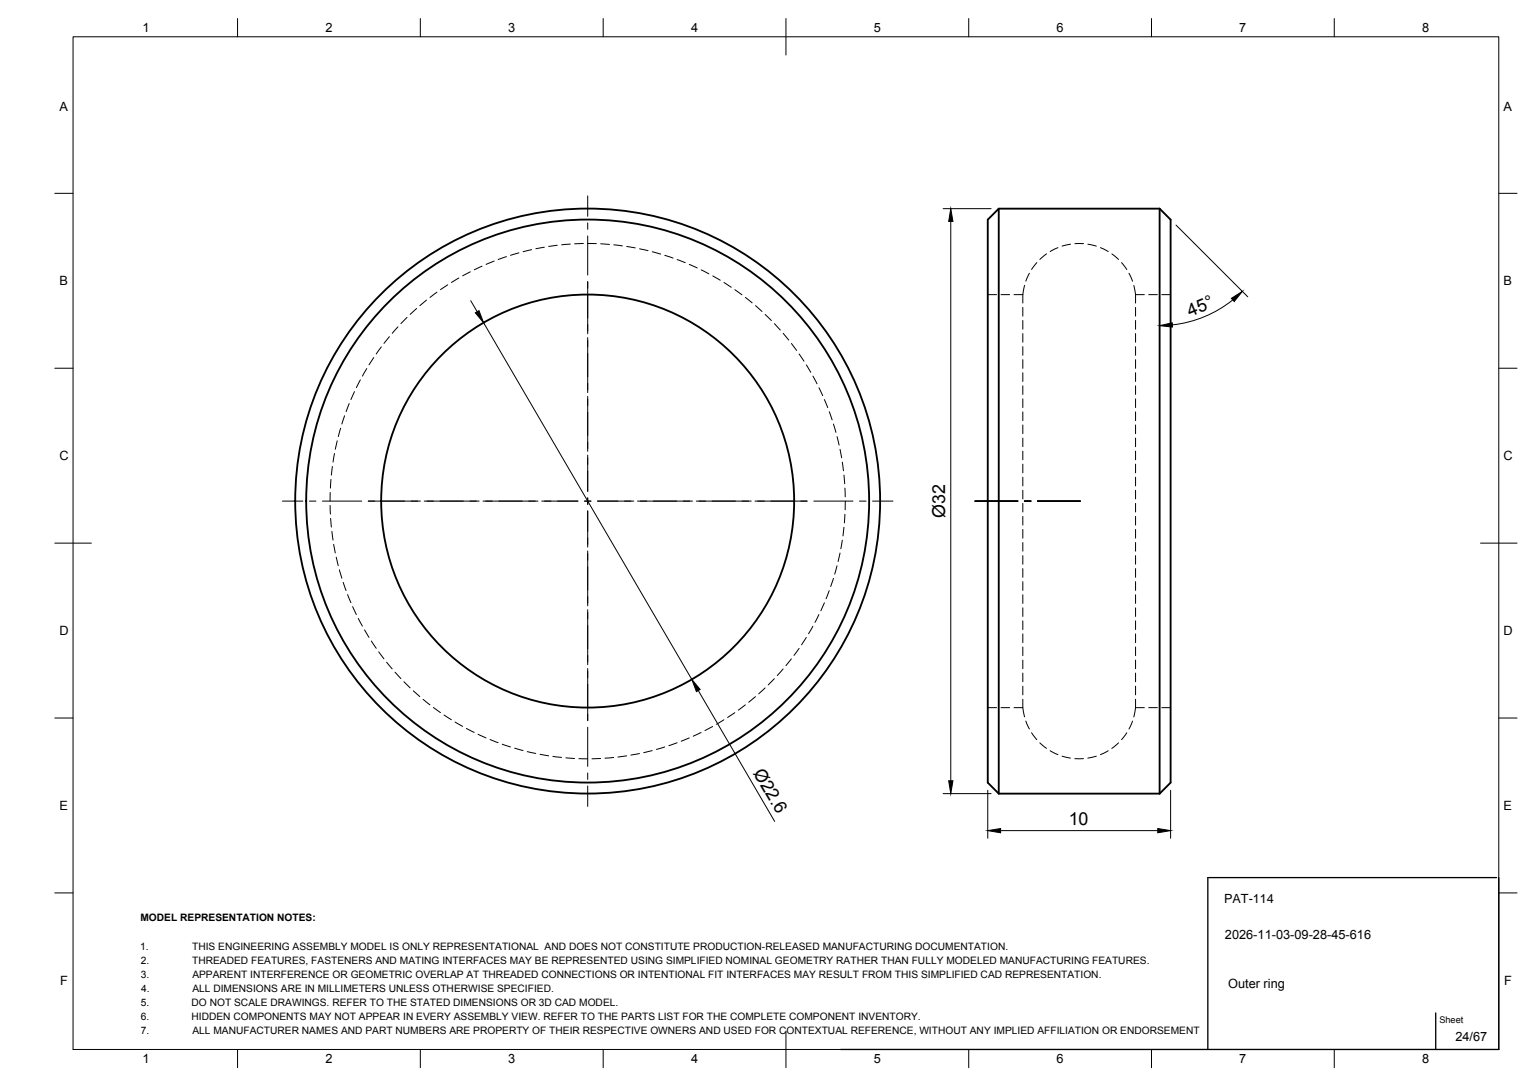
ISO-10303-21;
HEADER;
/* Generated by software containing ST-Developer
 * from STEP Tools, Inc. (www.steptools.com) 
 */

FILE_DESCRIPTION(
/* description */ ('Two-stage gear reducer in split housing'),
/* implementation_level */ '2;1');

FILE_NAME(
/* name */ 'Outer ring.step',
/* time_stamp */ '2026-10-28T03:22:31-07:00',
/* author */ (''),
/* organization */ (''),
/* preprocessor_version */ 'ST-DEVELOPER v20.2',
/* originating_system */ 'Autodesk Translation Framework v15.17.0.0',
/* authorisation */ '');

FILE_SCHEMA (('AUTOMOTIVE_DESIGN { 1 0 10303 214 3 1 1 }'));
ENDSEC;

DATA;
#10=MECHANICAL_DESIGN_GEOMETRIC_PRESENTATION_REPRESENTATION('',(#1252),#73366);
#1098=TOROIDAL_SURFACE('',#17438,1.1,0.309556);
#1106=CONICAL_SURFACE('',#17449,1.57,0.785398163397449);
#1107=CONICAL_SURFACE('',#17453,1.57,0.785398163397449);
#1140=SHAPE_REPRESENTATION_RELATIONSHIP('SRR','None',#73628,#1196);
#1196=ADVANCED_BREP_SHAPE_REPRESENTATION('',(#1322),#73324);
#1252=STYLED_ITEM('',(#73988),#1322);
#1322=MANIFOLD_SOLID_BREP('Body1',#16141);
#1521=FACE_BOUND('',#3371,.T.);
#1522=FACE_BOUND('',#3376,.T.);
#1757=PLANE('',#17446);
#1758=PLANE('',#17455);
#2308=FACE_OUTER_BOUND('',#3368,.T.);
#2309=FACE_OUTER_BOUND('',#3369,.T.);
#2310=FACE_OUTER_BOUND('',#3370,.T.);
#2311=FACE_OUTER_BOUND('',#3372,.T.);
#2312=FACE_OUTER_BOUND('',#3373,.T.);
#2313=FACE_OUTER_BOUND('',#3374,.T.);
#2314=FACE_OUTER_BOUND('',#3375,.T.);
#2315=FACE_OUTER_BOUND('',#3377,.T.);
#3368=EDGE_LOOP('',(#11847,#11848,#11849,#11850,#11851,#11852));
#3369=EDGE_LOOP('',(#11853,#11854,#11855,#11856,#11857));
#3370=EDGE_LOOP('',(#11858));
#3371=EDGE_LOOP('',(#11859));
#3372=EDGE_LOOP('',(#11860,#11861,#11862,#11863));
#3373=EDGE_LOOP('',(#11864,#11865,#11866,#11867));
#3374=EDGE_LOOP('',(#11868,#11869,#11870,#11871));
#3375=EDGE_LOOP('',(#11872));
#3376=EDGE_LOOP('',(#11873));
#3377=EDGE_LOOP('',(#11874,#11875,#11876,#11877,#11878));
#4428=LINE('',#24230,#5452);
#4429=LINE('',#24239,#5453);
#4430=LINE('',#24243,#5454);
#4431=LINE('',#24247,#5455);
#4432=LINE('',#24250,#5456);
#5452=VECTOR('',#20098,1.129765);
#5453=VECTOR('',#20109,1.57);
#5454=VECTOR('',#20114,1.6);
#5455=VECTOR('',#20119,1.57);
#5456=VECTOR('',#20124,1.129765);
#6402=CIRCLE('',#17439,1.129765);
#6403=CIRCLE('',#17440,1.129765);
#6404=CIRCLE('',#17441,0.309556);
#6405=CIRCLE('',#17442,1.129765);
#6406=CIRCLE('',#17443,1.129765);
#6407=CIRCLE('',#17445,1.129765);
#6408=CIRCLE('',#17447,1.54);
#6409=CIRCLE('',#17448,1.129765);
#6410=CIRCLE('',#17450,1.6);
#6411=CIRCLE('',#17452,1.6);
#6412=CIRCLE('',#17454,1.54);
#7269=VERTEX_POINT('',#24218);
#7270=VERTEX_POINT('',#24219);
#7271=VERTEX_POINT('',#24222);
#7272=VERTEX_POINT('',#24224);
#7273=VERTEX_POINT('',#24228);
#7274=VERTEX_POINT('',#24232);
#7275=VERTEX_POINT('',#24234);
#7276=VERTEX_POINT('',#24237);
#7277=VERTEX_POINT('',#24241);
#7278=VERTEX_POINT('',#24245);
#8977=EDGE_CURVE('',#7269,#7270,#6402,.T.);
#8978=EDGE_CURVE('',#7270,#7269,#6403,.T.);
#8979=EDGE_CURVE('',#7270,#7271,#6404,.T.);
#8980=EDGE_CURVE('',#7272,#7271,#6405,.T.);
#8981=EDGE_CURVE('',#7271,#7272,#6406,.T.);
#8982=EDGE_CURVE('',#7273,#7273,#6407,.T.);
#8983=EDGE_CURVE('',#7273,#7272,#4428,.T.);
#8984=EDGE_CURVE('',#7274,#7274,#6408,.T.);
#8985=EDGE_CURVE('',#7275,#7275,#6409,.T.);
#8986=EDGE_CURVE('',#7276,#7276,#6410,.T.);
#8987=EDGE_CURVE('',#7276,#7274,#4429,.T.);
#8988=EDGE_CURVE('',#7277,#7277,#6411,.T.);
#8989=EDGE_CURVE('',#7277,#7276,#4430,.T.);
#8990=EDGE_CURVE('',#7278,#7278,#6412,.T.);
#8991=EDGE_CURVE('',#7278,#7277,#4431,.T.);
#8992=EDGE_CURVE('',#7269,#7275,#4432,.T.);
#11847=ORIENTED_EDGE('',*,*,#8977,.F.);
#11848=ORIENTED_EDGE('',*,*,#8978,.F.);
#11849=ORIENTED_EDGE('',*,*,#8979,.T.);
#11850=ORIENTED_EDGE('',*,*,#8980,.F.);
#11851=ORIENTED_EDGE('',*,*,#8981,.F.);
#11852=ORIENTED_EDGE('',*,*,#8979,.F.);
#11853=ORIENTED_EDGE('',*,*,#8982,.T.);
#11854=ORIENTED_EDGE('',*,*,#8983,.T.);
#11855=ORIENTED_EDGE('',*,*,#8980,.T.);
#11856=ORIENTED_EDGE('',*,*,#8981,.T.);
#11857=ORIENTED_EDGE('',*,*,#8983,.F.);
#11858=ORIENTED_EDGE('',*,*,#8984,.F.);
#11859=ORIENTED_EDGE('',*,*,#8985,.T.);
#11860=ORIENTED_EDGE('',*,*,#8986,.F.);
#11861=ORIENTED_EDGE('',*,*,#8987,.T.);
#11862=ORIENTED_EDGE('',*,*,#8984,.T.);
#11863=ORIENTED_EDGE('',*,*,#8987,.F.);
#11864=ORIENTED_EDGE('',*,*,#8988,.F.);
#11865=ORIENTED_EDGE('',*,*,#8989,.T.);
#11866=ORIENTED_EDGE('',*,*,#8986,.T.);
#11867=ORIENTED_EDGE('',*,*,#8989,.F.);
#11868=ORIENTED_EDGE('',*,*,#8990,.F.);
#11869=ORIENTED_EDGE('',*,*,#8991,.T.);
#11870=ORIENTED_EDGE('',*,*,#8988,.T.);
#11871=ORIENTED_EDGE('',*,*,#8991,.F.);
#11872=ORIENTED_EDGE('',*,*,#8990,.T.);
#11873=ORIENTED_EDGE('',*,*,#8982,.F.);
#11874=ORIENTED_EDGE('',*,*,#8977,.T.);
#11875=ORIENTED_EDGE('',*,*,#8978,.T.);
#11876=ORIENTED_EDGE('',*,*,#8992,.T.);
#11877=ORIENTED_EDGE('',*,*,#8985,.F.);
#11878=ORIENTED_EDGE('',*,*,#8992,.F.);
#15052=CYLINDRICAL_SURFACE('',#17444,1.129765);
#15053=CYLINDRICAL_SURFACE('',#17451,1.6);
#15054=CYLINDRICAL_SURFACE('',#17456,1.129765);
#15515=ADVANCED_FACE('',(#2308),#1098,.F.);
#15516=ADVANCED_FACE('',(#2309),#15052,.F.);
#15517=ADVANCED_FACE('',(#2310,#1521),#1757,.T.);
#15518=ADVANCED_FACE('',(#2311),#1106,.T.);
#15519=ADVANCED_FACE('',(#2312),#15053,.T.);
#15520=ADVANCED_FACE('',(#2313),#1107,.T.);
#15521=ADVANCED_FACE('',(#2314,#1522),#1758,.T.);
#15522=ADVANCED_FACE('',(#2315),#15054,.F.);
#16141=CLOSED_SHELL('',(#15515,#15516,#15517,#15518,#15519,#15520,#15521,
#15522));
#17437=AXIS2_PLACEMENT_3D('',#24216,#20080,#20081);
#17438=AXIS2_PLACEMENT_3D('',#24217,#20082,#20083);
#17439=AXIS2_PLACEMENT_3D('',#24220,#20084,#20085);
#17440=AXIS2_PLACEMENT_3D('',#24221,#20086,#20087);
#17441=AXIS2_PLACEMENT_3D('',#24223,#20088,#20089);
#17442=AXIS2_PLACEMENT_3D('',#24225,#20090,#20091);
#17443=AXIS2_PLACEMENT_3D('',#24226,#20092,#20093);
#17444=AXIS2_PLACEMENT_3D('',#24227,#20094,#20095);
#17445=AXIS2_PLACEMENT_3D('',#24229,#20096,#20097);
#17446=AXIS2_PLACEMENT_3D('',#24231,#20099,#20100);
#17447=AXIS2_PLACEMENT_3D('',#24233,#20101,#20102);
#17448=AXIS2_PLACEMENT_3D('',#24235,#20103,#20104);
#17449=AXIS2_PLACEMENT_3D('',#24236,#20105,#20106);
#17450=AXIS2_PLACEMENT_3D('',#24238,#20107,#20108);
#17451=AXIS2_PLACEMENT_3D('',#24240,#20110,#20111);
#17452=AXIS2_PLACEMENT_3D('',#24242,#20112,#20113);
#17453=AXIS2_PLACEMENT_3D('',#24244,#20115,#20116);
#17454=AXIS2_PLACEMENT_3D('',#24246,#20117,#20118);
#17455=AXIS2_PLACEMENT_3D('',#24248,#20120,#20121);
#17456=AXIS2_PLACEMENT_3D('',#24249,#20122,#20123);
#20080=DIRECTION('axis',(0.,0.,1.));
#20081=DIRECTION('refdir',(1.,0.,0.));
#20082=DIRECTION('center_axis',(0.,-1.,0.));
#20083=DIRECTION('ref_axis',(0.,0.,-1.));
#20084=DIRECTION('center_axis',(0.,-1.,0.));
#20085=DIRECTION('ref_axis',(1.,0.,0.));
#20086=DIRECTION('center_axis',(0.,-1.,0.));
#20087=DIRECTION('ref_axis',(1.,0.,0.));
#20088=DIRECTION('center_axis',(1.,0.,1.22464679914735E-16));
#20089=DIRECTION('ref_axis',(-1.22464679914735E-16,0.,1.));
#20090=DIRECTION('center_axis',(0.,1.,0.));
#20091=DIRECTION('ref_axis',(1.,0.,0.));
#20092=DIRECTION('center_axis',(0.,1.,0.));
#20093=DIRECTION('ref_axis',(1.,0.,0.));
#20094=DIRECTION('center_axis',(0.,-1.,0.));
#20095=DIRECTION('ref_axis',(1.,0.,0.));
#20096=DIRECTION('center_axis',(0.,-1.,0.));
#20097=DIRECTION('ref_axis',(1.,0.,0.));
#20098=DIRECTION('',(0.,1.,0.));
#20099=DIRECTION('center_axis',(0.,1.,0.));
#20100=DIRECTION('ref_axis',(0.,0.,1.));
#20101=DIRECTION('center_axis',(0.,-1.,0.));
#20102=DIRECTION('ref_axis',(1.,0.,0.));
#20103=DIRECTION('center_axis',(0.,-1.,0.));
#20104=DIRECTION('ref_axis',(1.,0.,0.));
#20105=DIRECTION('center_axis',(0.,-1.,0.));
#20106=DIRECTION('ref_axis',(1.,0.,0.));
#20107=DIRECTION('center_axis',(0.,-1.,0.));
#20108=DIRECTION('ref_axis',(1.,0.,0.));
#20109=DIRECTION('',(0.707106781186548,0.707106781186547,8.65956056235494E-17));
#20110=DIRECTION('center_axis',(0.,-1.,0.));
#20111=DIRECTION('ref_axis',(1.,0.,0.));
#20112=DIRECTION('center_axis',(0.,-1.,0.));
#20113=DIRECTION('ref_axis',(1.,0.,0.));
#20114=DIRECTION('',(0.,1.,0.));
#20115=DIRECTION('center_axis',(0.,1.,0.));
#20116=DIRECTION('ref_axis',(1.,0.,0.));
#20117=DIRECTION('center_axis',(0.,-1.,0.));
#20118=DIRECTION('ref_axis',(1.,0.,0.));
#20119=DIRECTION('',(-0.707106781186548,0.707106781186547,-8.65956056235494E-17));
#20120=DIRECTION('center_axis',(0.,-1.,0.));
#20121=DIRECTION('ref_axis',(0.,0.,-1.));
#20122=DIRECTION('center_axis',(0.,-1.,0.));
#20123=DIRECTION('ref_axis',(1.,0.,0.));
#20124=DIRECTION('',(0.,1.,0.));
#24216=CARTESIAN_POINT('',(0.,0.,0.));
#24217=CARTESIAN_POINT('Origin',(0.,0.,0.));
#24218=CARTESIAN_POINT('',(-1.129765,0.308121667383195,-1.38356309103871E-16));
#24219=CARTESIAN_POINT('',(-1.38356309103871E-16,0.308121667383195,1.129765));
#24220=CARTESIAN_POINT('Origin',(0.,0.308121667383195,0.));
#24221=CARTESIAN_POINT('Origin',(0.,0.308121667383195,0.));
#24222=CARTESIAN_POINT('',(-1.38356309103871E-16,-0.308121667383195,1.129765));
#24223=CARTESIAN_POINT('Origin',(-1.34711147906209E-16,0.,1.1));
#24224=CARTESIAN_POINT('',(-1.129765,-0.308121667383195,1.38356309103871E-16));
#24225=CARTESIAN_POINT('Origin',(0.,-0.308121667383195,0.));
#24226=CARTESIAN_POINT('Origin',(0.,-0.308121667383195,0.));
#24227=CARTESIAN_POINT('Origin',(0.,0.,0.));
#24228=CARTESIAN_POINT('',(-1.129765,-0.5,-1.38356309103871E-16));
#24229=CARTESIAN_POINT('Origin',(0.,-0.5,0.));
#24230=CARTESIAN_POINT('',(-1.129765,0.,-1.38356309103871E-16));
#24231=CARTESIAN_POINT('Origin',(1.54,0.5,0.));
#24232=CARTESIAN_POINT('',(-1.54,0.5,-1.88595607068692E-16));
#24233=CARTESIAN_POINT('Origin',(0.,0.5,0.));
#24234=CARTESIAN_POINT('',(-1.129765,0.5,-1.38356309103871E-16));
#24235=CARTESIAN_POINT('Origin',(0.,0.5,0.));
#24236=CARTESIAN_POINT('Origin',(0.,0.47,0.));
#24237=CARTESIAN_POINT('',(-1.6,0.44,-1.95943487863577E-16));
#24238=CARTESIAN_POINT('Origin',(0.,0.44,0.));
#24239=CARTESIAN_POINT('',(-1.57,0.47,-1.92269547466134E-16));
#24240=CARTESIAN_POINT('Origin',(0.,0.,0.));
#24241=CARTESIAN_POINT('',(-1.6,-0.44,-1.95943487863577E-16));
#24242=CARTESIAN_POINT('Origin',(0.,-0.44,0.));
#24243=CARTESIAN_POINT('',(-1.6,0.,-1.95943487863577E-16));
#24244=CARTESIAN_POINT('Origin',(0.,-0.47,0.));
#24245=CARTESIAN_POINT('',(-1.54,-0.5,-1.88595607068692E-16));
#24246=CARTESIAN_POINT('Origin',(0.,-0.5,0.));
#24247=CARTESIAN_POINT('',(-1.57,-0.47,-1.92269547466134E-16));
#24248=CARTESIAN_POINT('Origin',(1.129765,-0.5,0.));
#24249=CARTESIAN_POINT('Origin',(0.,0.,0.));
#24250=CARTESIAN_POINT('',(-1.129765,0.,-1.38356309103871E-16));
#73260=UNCERTAINTY_MEASURE_WITH_UNIT(LENGTH_MEASURE(0.001),#73367,
'DISTANCE_ACCURACY_VALUE',
'Maximum model space distance between geometric entities at asserted c
onnectivities');
#73302=UNCERTAINTY_MEASURE_WITH_UNIT(LENGTH_MEASURE(0.001),#73367,
'DISTANCE_ACCURACY_VALUE',
'Maximum model space distance between geometric entities at asserted c
onnectivities');
#73324=(
GEOMETRIC_REPRESENTATION_CONTEXT(3)
GLOBAL_UNCERTAINTY_ASSIGNED_CONTEXT((#73260))
GLOBAL_UNIT_ASSIGNED_CONTEXT((#73367,#73369,#73370))
REPRESENTATION_CONTEXT('','3D')
);
#73366=(
GEOMETRIC_REPRESENTATION_CONTEXT(3)
GLOBAL_UNCERTAINTY_ASSIGNED_CONTEXT((#73302))
GLOBAL_UNIT_ASSIGNED_CONTEXT((#73367,#73369,#73370))
REPRESENTATION_CONTEXT('','3D')
);
#73367=(
LENGTH_UNIT()
NAMED_UNIT(*)
SI_UNIT(.CENTI.,.METRE.)
);
#73369=(
NAMED_UNIT(*)
PLANE_ANGLE_UNIT()
SI_UNIT($,.RADIAN.)
);
#73370=(
NAMED_UNIT(*)
SI_UNIT($,.STERADIAN.)
SOLID_ANGLE_UNIT()
);
#73392=SHAPE_DEFINITION_REPRESENTATION(#73455,#73628);
#73455=PRODUCT_DEFINITION_SHAPE('',$,#73692);
#73628=SHAPE_REPRESENTATION('',(#17437),#73324);
#73670=PRODUCT_DEFINITION_CONTEXT('part definition',#73861,'design');
#73692=PRODUCT_DEFINITION('Outer ring','Outer ring',#73755,#73670);
#73755=PRODUCT_DEFINITION_FORMATION('',$,#73884);
#73861=APPLICATION_CONTEXT(
'Core Data for Automotive Mechanical Design Process');
#73862=PRODUCT_CONTEXT('part definition',#73861,'mechanical');
#73884=PRODUCT('Outer ring','Outer ring','Outer ring',(#73862));
#73982=COLOUR_RGB('Grey',0.48,0.52,0.57);
#73983=FILL_AREA_STYLE_COLOUR('',#73982);
#73984=FILL_AREA_STYLE('',(#73983));
#73985=SURFACE_STYLE_FILL_AREA(#73984);
#73986=SURFACE_SIDE_STYLE('',(#73985));
#73987=SURFACE_STYLE_USAGE(.BOTH.,#73986);
#73988=PRESENTATION_STYLE_ASSIGNMENT((#73987));
ENDSEC;
END-ISO-10303-21;
